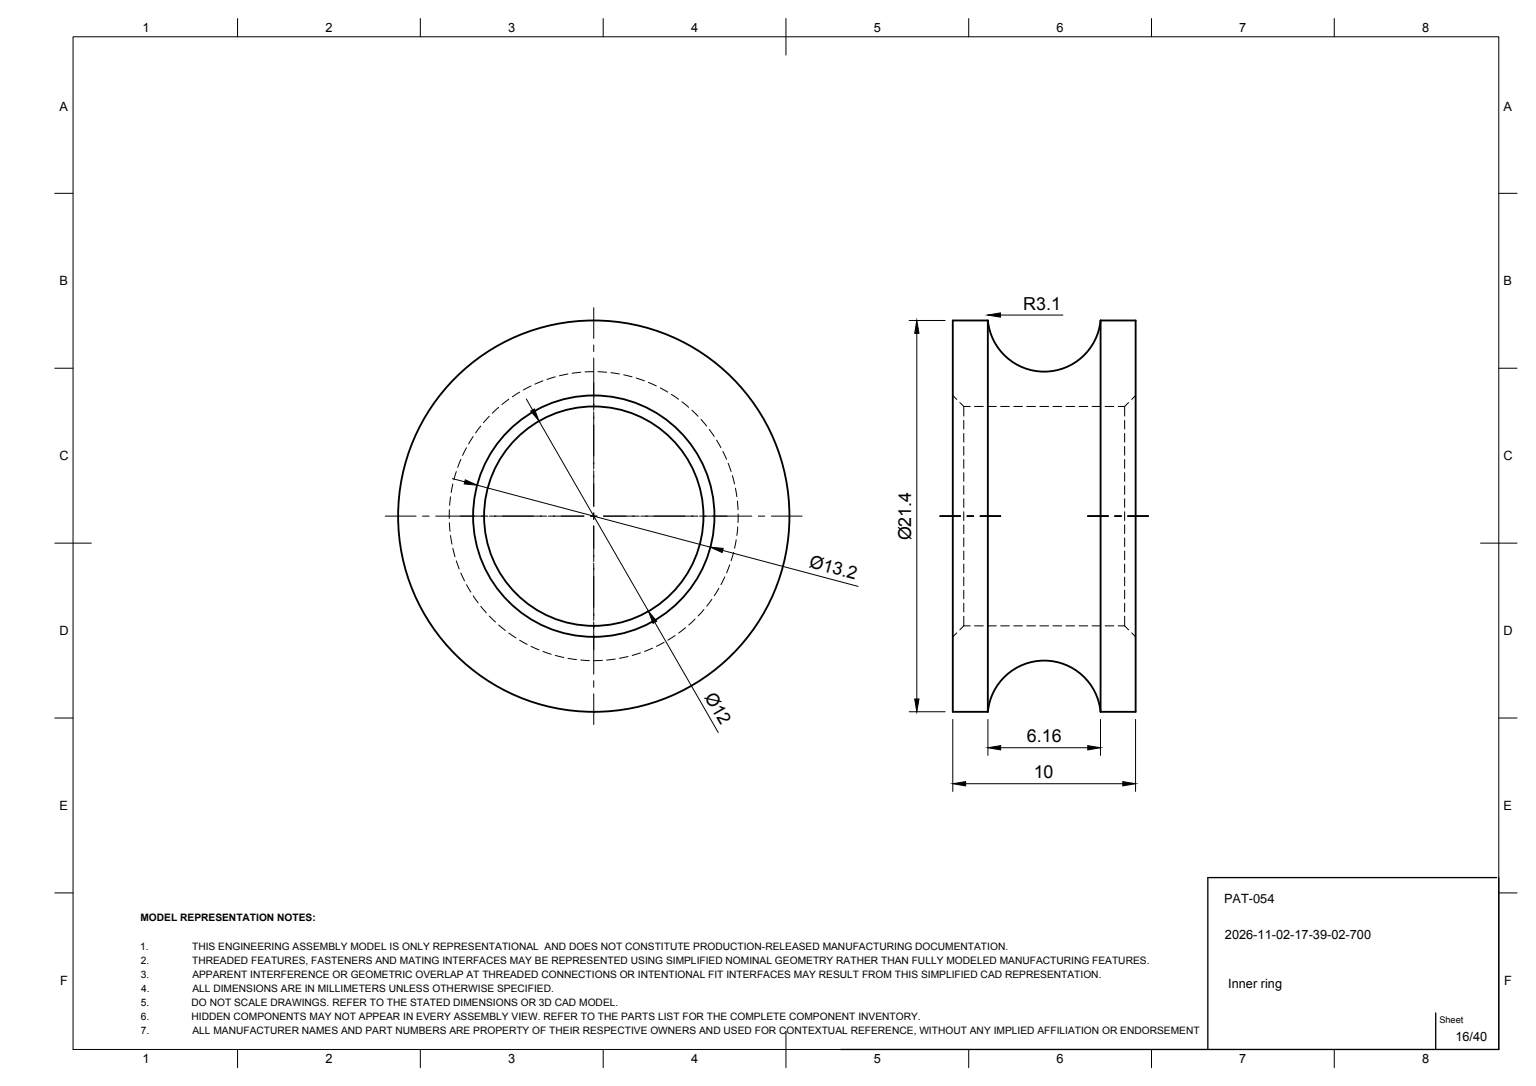
ISO-10303-21;
HEADER;
/* Generated by software containing ST-Developer
 * from STEP Tools, Inc. (www.steptools.com) 
 */

FILE_DESCRIPTION(
/* description */ ('PAT-054'),
/* implementation_level */ '2;1');

FILE_NAME(
/* name */ 'Inner ring.step',
/* time_stamp */ '2026-10-29T16:38:13-07:00',
/* author */ (''),
/* organization */ (''),
/* preprocessor_version */ 'ST-DEVELOPER v20.2',
/* originating_system */ 'Autodesk Translation Framework v15.17.0.0',
/* authorisation */ '');

FILE_SCHEMA (('AUTOMOTIVE_DESIGN { 1 0 10303 214 3 1 1 }'));
ENDSEC;

DATA;
#10=MECHANICAL_DESIGN_GEOMETRIC_PRESENTATION_REPRESENTATION('',(#908),#33981);
#777=CONICAL_SURFACE('',#13884,0.63,0.785398163397448);
#778=CONICAL_SURFACE('',#13891,0.63,0.785398163397448);
#807=TOROIDAL_SURFACE('',#13873,1.1,0.309556);
#820=SHAPE_REPRESENTATION_RELATIONSHIP('SRR','None',#34194,#864);
#864=ADVANCED_BREP_SHAPE_REPRESENTATION('',(#967),#33942);
#908=STYLED_ITEM('',(#34517),#967);
#967=MANIFOLD_SOLID_BREP('Body1',#13019);
#1128=FACE_BOUND('',#2572,.T.);
#1129=FACE_BOUND('',#2575,.T.);
#1311=PLANE('',#13886);
#1312=PLANE('',#13889);
#1728=FACE_OUTER_BOUND('',#2567,.T.);
#1729=FACE_OUTER_BOUND('',#2568,.T.);
#1730=FACE_OUTER_BOUND('',#2569,.T.);
#1731=FACE_OUTER_BOUND('',#2570,.T.);
#1732=FACE_OUTER_BOUND('',#2571,.T.);
#1733=FACE_OUTER_BOUND('',#2573,.T.);
#1734=FACE_OUTER_BOUND('',#2574,.T.);
#1735=FACE_OUTER_BOUND('',#2576,.T.);
#2567=EDGE_LOOP('',(#9227,#9228,#9229,#9230,#9231,#9232));
#2568=EDGE_LOOP('',(#9233,#9234,#9235,#9236,#9237));
#2569=EDGE_LOOP('',(#9238,#9239,#9240,#9241));
#2570=EDGE_LOOP('',(#9242,#9243,#9244,#9245));
#2571=EDGE_LOOP('',(#9246));
#2572=EDGE_LOOP('',(#9247));
#2573=EDGE_LOOP('',(#9248,#9249,#9250,#9251,#9252));
#2574=EDGE_LOOP('',(#9253));
#2575=EDGE_LOOP('',(#9254));
#2576=EDGE_LOOP('',(#9255,#9256,#9257,#9258));
#3458=LINE('',#19279,#4392);
#3459=LINE('',#19285,#4393);
#3460=LINE('',#19289,#4394);
#3461=LINE('',#19295,#4395);
#3462=LINE('',#19300,#4396);
#4392=VECTOR('',#15753,1.070235);
#4393=VECTOR('',#15760,0.6);
#4394=VECTOR('',#15765,0.63);
#4395=VECTOR('',#15774,1.070235);
#4396=VECTOR('',#15781,0.63);
#5253=CIRCLE('',#13874,1.070235);
#5254=CIRCLE('',#13875,1.070235);
#5255=CIRCLE('',#13876,0.309556);
#5256=CIRCLE('',#13877,1.070235);
#5257=CIRCLE('',#13878,1.070235);
#5258=CIRCLE('',#13880,1.070235);
#5259=CIRCLE('',#13882,0.6);
#5260=CIRCLE('',#13883,0.6);
#5261=CIRCLE('',#13885,0.66);
#5262=CIRCLE('',#13888,1.070235);
#5263=CIRCLE('',#13890,0.66);
#5816=VERTEX_POINT('',#19268);
#5817=VERTEX_POINT('',#19269);
#5818=VERTEX_POINT('',#19272);
#5819=VERTEX_POINT('',#19274);
#5820=VERTEX_POINT('',#19278);
#5821=VERTEX_POINT('',#19282);
#5822=VERTEX_POINT('',#19284);
#5823=VERTEX_POINT('',#19288);
#5824=VERTEX_POINT('',#19293);
#5825=VERTEX_POINT('',#19297);
#7113=EDGE_CURVE('',#5816,#5817,#5253,.T.);
#7114=EDGE_CURVE('',#5817,#5816,#5254,.T.);
#7115=EDGE_CURVE('',#5817,#5818,#5255,.T.);
#7116=EDGE_CURVE('',#5819,#5818,#5256,.T.);
#7117=EDGE_CURVE('',#5818,#5819,#5257,.T.);
#7118=EDGE_CURVE('',#5819,#5820,#3458,.T.);
#7119=EDGE_CURVE('',#5820,#5820,#5258,.T.);
#7120=EDGE_CURVE('',#5821,#5821,#5259,.T.);
#7121=EDGE_CURVE('',#5821,#5822,#3459,.T.);
#7122=EDGE_CURVE('',#5822,#5822,#5260,.T.);
#7123=EDGE_CURVE('',#5822,#5823,#3460,.T.);
#7124=EDGE_CURVE('',#5823,#5823,#5261,.T.);
#7125=EDGE_CURVE('',#5824,#5824,#5262,.T.);
#7126=EDGE_CURVE('',#5824,#5816,#3461,.T.);
#7127=EDGE_CURVE('',#5825,#5825,#5263,.T.);
#7128=EDGE_CURVE('',#5825,#5821,#3462,.T.);
#9227=ORIENTED_EDGE('',*,*,#7113,.F.);
#9228=ORIENTED_EDGE('',*,*,#7114,.F.);
#9229=ORIENTED_EDGE('',*,*,#7115,.T.);
#9230=ORIENTED_EDGE('',*,*,#7116,.F.);
#9231=ORIENTED_EDGE('',*,*,#7117,.F.);
#9232=ORIENTED_EDGE('',*,*,#7115,.F.);
#9233=ORIENTED_EDGE('',*,*,#7116,.T.);
#9234=ORIENTED_EDGE('',*,*,#7117,.T.);
#9235=ORIENTED_EDGE('',*,*,#7118,.T.);
#9236=ORIENTED_EDGE('',*,*,#7119,.T.);
#9237=ORIENTED_EDGE('',*,*,#7118,.F.);
#9238=ORIENTED_EDGE('',*,*,#7120,.T.);
#9239=ORIENTED_EDGE('',*,*,#7121,.T.);
#9240=ORIENTED_EDGE('',*,*,#7122,.F.);
#9241=ORIENTED_EDGE('',*,*,#7121,.F.);
#9242=ORIENTED_EDGE('',*,*,#7122,.T.);
#9243=ORIENTED_EDGE('',*,*,#7123,.T.);
#9244=ORIENTED_EDGE('',*,*,#7124,.F.);
#9245=ORIENTED_EDGE('',*,*,#7123,.F.);
#9246=ORIENTED_EDGE('',*,*,#7119,.F.);
#9247=ORIENTED_EDGE('',*,*,#7124,.T.);
#9248=ORIENTED_EDGE('',*,*,#7125,.F.);
#9249=ORIENTED_EDGE('',*,*,#7126,.T.);
#9250=ORIENTED_EDGE('',*,*,#7113,.T.);
#9251=ORIENTED_EDGE('',*,*,#7114,.T.);
#9252=ORIENTED_EDGE('',*,*,#7126,.F.);
#9253=ORIENTED_EDGE('',*,*,#7125,.T.);
#9254=ORIENTED_EDGE('',*,*,#7127,.F.);
#9255=ORIENTED_EDGE('',*,*,#7127,.T.);
#9256=ORIENTED_EDGE('',*,*,#7128,.T.);
#9257=ORIENTED_EDGE('',*,*,#7120,.F.);
#9258=ORIENTED_EDGE('',*,*,#7128,.F.);
#12049=CYLINDRICAL_SURFACE('',#13879,1.070235);
#12050=CYLINDRICAL_SURFACE('',#13881,0.6);
#12051=CYLINDRICAL_SURFACE('',#13887,1.070235);
#12440=ADVANCED_FACE('',(#1728),#807,.F.);
#12441=ADVANCED_FACE('',(#1729),#12049,.T.);
#12442=ADVANCED_FACE('',(#1730),#12050,.F.);
#12443=ADVANCED_FACE('',(#1731),#777,.F.);
#12444=ADVANCED_FACE('',(#1732,#1128),#1311,.T.);
#12445=ADVANCED_FACE('',(#1733),#12051,.T.);
#12446=ADVANCED_FACE('',(#1734,#1129),#1312,.T.);
#12447=ADVANCED_FACE('',(#1735),#778,.F.);
#13019=CLOSED_SHELL('',(#12440,#12441,#12442,#12443,#12444,#12445,#12446,
#12447));
#13872=AXIS2_PLACEMENT_3D('',#19266,#15737,#15738);
#13873=AXIS2_PLACEMENT_3D('',#19267,#15739,#15740);
#13874=AXIS2_PLACEMENT_3D('',#19270,#15741,#15742);
#13875=AXIS2_PLACEMENT_3D('',#19271,#15743,#15744);
#13876=AXIS2_PLACEMENT_3D('',#19273,#15745,#15746);
#13877=AXIS2_PLACEMENT_3D('',#19275,#15747,#15748);
#13878=AXIS2_PLACEMENT_3D('',#19276,#15749,#15750);
#13879=AXIS2_PLACEMENT_3D('',#19277,#15751,#15752);
#13880=AXIS2_PLACEMENT_3D('',#19280,#15754,#15755);
#13881=AXIS2_PLACEMENT_3D('',#19281,#15756,#15757);
#13882=AXIS2_PLACEMENT_3D('',#19283,#15758,#15759);
#13883=AXIS2_PLACEMENT_3D('',#19286,#15761,#15762);
#13884=AXIS2_PLACEMENT_3D('',#19287,#15763,#15764);
#13885=AXIS2_PLACEMENT_3D('',#19290,#15766,#15767);
#13886=AXIS2_PLACEMENT_3D('',#19291,#15768,#15769);
#13887=AXIS2_PLACEMENT_3D('',#19292,#15770,#15771);
#13888=AXIS2_PLACEMENT_3D('',#19294,#15772,#15773);
#13889=AXIS2_PLACEMENT_3D('',#19296,#15775,#15776);
#13890=AXIS2_PLACEMENT_3D('',#19298,#15777,#15778);
#13891=AXIS2_PLACEMENT_3D('',#19299,#15779,#15780);
#15737=DIRECTION('axis',(0.,0.,1.));
#15738=DIRECTION('refdir',(1.,0.,0.));
#15739=DIRECTION('center_axis',(0.,-1.,0.));
#15740=DIRECTION('ref_axis',(0.,0.,-1.));
#15741=DIRECTION('center_axis',(0.,-1.,0.));
#15742=DIRECTION('ref_axis',(1.,0.,0.));
#15743=DIRECTION('center_axis',(0.,-1.,0.));
#15744=DIRECTION('ref_axis',(1.,0.,0.));
#15745=DIRECTION('center_axis',(1.,0.,1.22464679914735E-16));
#15746=DIRECTION('ref_axis',(-1.22464679914735E-16,0.,1.));
#15747=DIRECTION('center_axis',(0.,1.,0.));
#15748=DIRECTION('ref_axis',(1.,0.,0.));
#15749=DIRECTION('center_axis',(0.,1.,0.));
#15750=DIRECTION('ref_axis',(1.,0.,0.));
#15751=DIRECTION('center_axis',(0.,-1.,0.));
#15752=DIRECTION('ref_axis',(1.,0.,0.));
#15753=DIRECTION('',(0.,1.,0.));
#15754=DIRECTION('center_axis',(0.,-1.,0.));
#15755=DIRECTION('ref_axis',(1.,0.,0.));
#15756=DIRECTION('center_axis',(0.,-1.,0.));
#15757=DIRECTION('ref_axis',(1.,0.,0.));
#15758=DIRECTION('center_axis',(0.,-1.,0.));
#15759=DIRECTION('ref_axis',(1.,0.,0.));
#15760=DIRECTION('',(0.,1.,0.));
#15761=DIRECTION('center_axis',(0.,-1.,0.));
#15762=DIRECTION('ref_axis',(1.,0.,0.));
#15763=DIRECTION('center_axis',(0.,1.,0.));
#15764=DIRECTION('ref_axis',(1.,0.,0.));
#15765=DIRECTION('',(-0.707106781186548,0.707106781186547,-8.65956056235493E-17));
#15766=DIRECTION('center_axis',(0.,-1.,0.));
#15767=DIRECTION('ref_axis',(1.,0.,0.));
#15768=DIRECTION('center_axis',(0.,1.,0.));
#15769=DIRECTION('ref_axis',(0.,0.,1.));
#15770=DIRECTION('center_axis',(0.,-1.,0.));
#15771=DIRECTION('ref_axis',(1.,0.,0.));
#15772=DIRECTION('center_axis',(0.,-1.,0.));
#15773=DIRECTION('ref_axis',(1.,0.,0.));
#15774=DIRECTION('',(0.,1.,0.));
#15775=DIRECTION('center_axis',(0.,-1.,0.));
#15776=DIRECTION('ref_axis',(0.,0.,-1.));
#15777=DIRECTION('center_axis',(0.,-1.,0.));
#15778=DIRECTION('ref_axis',(1.,0.,0.));
#15779=DIRECTION('center_axis',(0.,-1.,0.));
#15780=DIRECTION('ref_axis',(1.,0.,0.));
#15781=DIRECTION('',(0.707106781186548,0.707106781186547,8.65956056235493E-17));
#19266=CARTESIAN_POINT('',(0.,0.,0.));
#19267=CARTESIAN_POINT('Origin',(0.,0.,0.));
#19268=CARTESIAN_POINT('',(-1.070235,-0.308121667383195,-1.31065986708547E-16));
#19269=CARTESIAN_POINT('',(-1.31065986708547E-16,-0.308121667383195,1.070235));
#19270=CARTESIAN_POINT('Origin',(0.,-0.308121667383195,0.));
#19271=CARTESIAN_POINT('Origin',(0.,-0.308121667383195,0.));
#19272=CARTESIAN_POINT('',(-1.31065986708547E-16,0.308121667383195,1.070235));
#19273=CARTESIAN_POINT('Origin',(-1.34711147906209E-16,0.,1.1));
#19274=CARTESIAN_POINT('',(-1.070235,0.308121667383195,1.31065986708547E-16));
#19275=CARTESIAN_POINT('Origin',(0.,0.308121667383195,0.));
#19276=CARTESIAN_POINT('Origin',(0.,0.308121667383195,0.));
#19277=CARTESIAN_POINT('Origin',(0.,0.,0.));
#19278=CARTESIAN_POINT('',(-1.070235,0.5,-1.31065986708547E-16));
#19279=CARTESIAN_POINT('',(-1.070235,0.,-1.31065986708547E-16));
#19280=CARTESIAN_POINT('Origin',(0.,0.5,0.));
#19281=CARTESIAN_POINT('Origin',(0.,0.,0.));
#19282=CARTESIAN_POINT('',(-0.6,-0.44,-7.34788079488412E-17));
#19283=CARTESIAN_POINT('Origin',(0.,-0.44,0.));
#19284=CARTESIAN_POINT('',(-0.6,0.44,-7.34788079488412E-17));
#19285=CARTESIAN_POINT('',(-0.6,0.,-7.34788079488412E-17));
#19286=CARTESIAN_POINT('Origin',(0.,0.44,0.));
#19287=CARTESIAN_POINT('Origin',(0.,0.47,0.));
#19288=CARTESIAN_POINT('',(-0.66,0.5,-8.08266887437253E-17));
#19289=CARTESIAN_POINT('',(-0.63,0.47,-7.71527483462832E-17));
#19290=CARTESIAN_POINT('Origin',(0.,0.5,0.));
#19291=CARTESIAN_POINT('Origin',(1.070235,0.5,0.));
#19292=CARTESIAN_POINT('Origin',(0.,0.,0.));
#19293=CARTESIAN_POINT('',(-1.070235,-0.5,-1.31065986708547E-16));
#19294=CARTESIAN_POINT('Origin',(0.,-0.5,0.));
#19295=CARTESIAN_POINT('',(-1.070235,0.,-1.31065986708547E-16));
#19296=CARTESIAN_POINT('Origin',(0.66,-0.5,0.));
#19297=CARTESIAN_POINT('',(-0.66,-0.5,-8.08266887437253E-17));
#19298=CARTESIAN_POINT('Origin',(0.,-0.5,0.));
#19299=CARTESIAN_POINT('Origin',(0.,-0.47,0.));
#19300=CARTESIAN_POINT('',(-0.63,-0.47,-7.71527483462832E-17));
#33890=UNCERTAINTY_MEASURE_WITH_UNIT(LENGTH_MEASURE(0.001),#33982,
'DISTANCE_ACCURACY_VALUE',
'Maximum model space distance between geometric entities at asserted c
onnectivities');
#33929=UNCERTAINTY_MEASURE_WITH_UNIT(LENGTH_MEASURE(0.001),#33982,
'DISTANCE_ACCURACY_VALUE',
'Maximum model space distance between geometric entities at asserted c
onnectivities');
#33942=(
GEOMETRIC_REPRESENTATION_CONTEXT(3)
GLOBAL_UNCERTAINTY_ASSIGNED_CONTEXT((#33890))
GLOBAL_UNIT_ASSIGNED_CONTEXT((#33982,#33984,#33985))
REPRESENTATION_CONTEXT('','3D')
);
#33981=(
GEOMETRIC_REPRESENTATION_CONTEXT(3)
GLOBAL_UNCERTAINTY_ASSIGNED_CONTEXT((#33929))
GLOBAL_UNIT_ASSIGNED_CONTEXT((#33982,#33984,#33985))
REPRESENTATION_CONTEXT('','3D')
);
#33982=(
LENGTH_UNIT()
NAMED_UNIT(*)
SI_UNIT(.CENTI.,.METRE.)
);
#33984=(
NAMED_UNIT(*)
PLANE_ANGLE_UNIT()
SI_UNIT($,.RADIAN.)
);
#33985=(
NAMED_UNIT(*)
SI_UNIT($,.STERADIAN.)
SOLID_ANGLE_UNIT()
);
#33998=SHAPE_DEFINITION_REPRESENTATION(#34049,#34194);
#34049=PRODUCT_DEFINITION_SHAPE('',$,#34246);
#34194=SHAPE_REPRESENTATION('',(#13872),#33942);
#34233=PRODUCT_DEFINITION_CONTEXT('part definition',#34388,'design');
#34246=PRODUCT_DEFINITION('Inner ring','Inner ring',#34297,#34233);
#34297=PRODUCT_DEFINITION_FORMATION('',$,#34402);
#34388=APPLICATION_CONTEXT(
'Core Data for Automotive Mechanical Design Process');
#34389=PRODUCT_CONTEXT('part definition',#34388,'mechanical');
#34402=PRODUCT('Inner ring','Inner ring','Inner ring',(#34389));
#34511=COLOUR_RGB('Grey',0.48,0.52,0.57);
#34512=FILL_AREA_STYLE_COLOUR('',#34511);
#34513=FILL_AREA_STYLE('',(#34512));
#34514=SURFACE_STYLE_FILL_AREA(#34513);
#34515=SURFACE_SIDE_STYLE('',(#34514));
#34516=SURFACE_STYLE_USAGE(.BOTH.,#34515);
#34517=PRESENTATION_STYLE_ASSIGNMENT((#34516));
ENDSEC;
END-ISO-10303-21;
